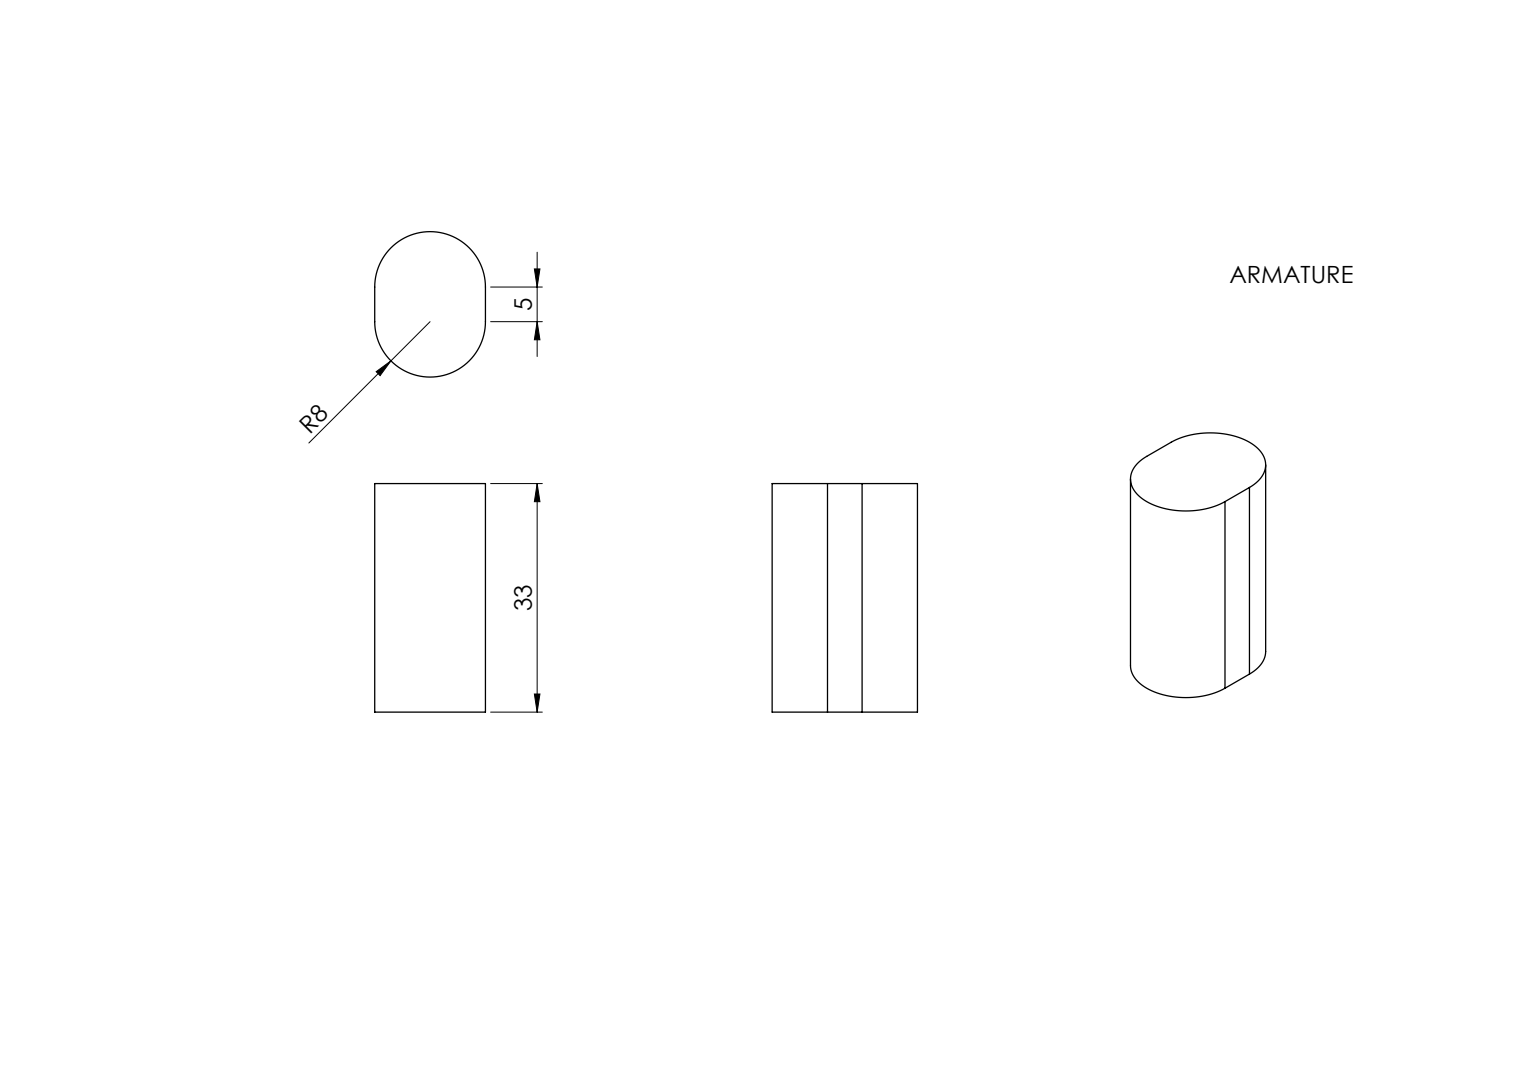
ISO-10303-21;
HEADER;
FILE_DESCRIPTION (('STEP AP214'),
    '1' );
FILE_NAME ('armature.step',
    '2026-10-25T16:39:07',
    ( '' ),
    ( '' ),
    'SwSTEP 2.0',
    'SolidWorks 2026',
    '' );
FILE_SCHEMA (( 'AUTOMOTIVE_DESIGN' ));
ENDSEC;

DATA;
#70=EDGE_LOOP ( 'NONE', ( #14455, #11089, #12235, #9427, #6688 ) ) ;
#196=VERTEX_POINT ( 'NONE', #13765 ) ;
#256=CARTESIAN_POINT ( 'NONE',  ( 7.960204194457794491E-16, 43.00000000000000000, 6.499999999999999112 ) ) ;
#309=AXIS2_PLACEMENT_3D ( 'NONE', #1703, #12902, #17104 ) ;
#401=CARTESIAN_POINT ( 'NONE',  ( 0.000000000000000000, 43.00000000000000000, -6.499999999999999112 ) ) ;
#459=( NAMED_UNIT ( * ) PLANE_ANGLE_UNIT ( ) SI_UNIT ( $, .RADIAN. ) );
#592=EDGE_CURVE ( 'NONE', #196, #11177, #4131, .T. ) ;
#631=EDGE_LOOP ( 'NONE', ( #5395, #16207, #13707, #2530 ) ) ;
#732=DIRECTION ( 'NONE',  ( 0.000000000000000000, 1.000000000000000000, 0.000000000000000000 ) ) ;
#736=DIRECTION ( 'NONE',  ( 0.000000000000000000, 0.000000000000000000, -1.000000000000000000 ) ) ;
#757=EDGE_LOOP ( 'NONE', ( #3139, #14699 ) ) ;
#760=FACE_OUTER_BOUND ( 'NONE', #70, .T. ) ;
#909=EDGE_CURVE ( 'NONE', #2259, #4661, #14792, .T. ) ;
#919=SURFACE_STYLE_USAGE ( .BOTH. , #14844 ) ;
#953=CIRCLE ( 'NONE', #984, 8.000000000000000000 ) ;
#956=( GEOMETRIC_REPRESENTATION_CONTEXT ( 3 ) GLOBAL_UNCERTAINTY_ASSIGNED_CONTEXT ( ( #17928 ) ) GLOBAL_UNIT_ASSIGNED_CONTEXT ( ( #7948, #17991, #15201 ) ) REPRESENTATION_CONTEXT ( 'NONE', 'WORKASPACE' ) );
#984=AXIS2_PLACEMENT_3D ( 'NONE', #4156, #12407, #11016 ) ;
#1007=DIRECTION ( 'NONE',  ( -0.000000000000000000, -1.000000000000000000, -0.000000000000000000 ) ) ;
#1011=ORIENTED_EDGE ( 'NONE', *, *, #17505, .F. ) ;
#1041=ORIENTED_EDGE ( 'NONE', *, *, #17682, .F. ) ;
#1082=LINE ( 'NONE', #2294, #16709 ) ;
#1153=DIRECTION ( 'NONE',  ( 0.000000000000000000, 1.000000000000000000, 0.000000000000000000 ) ) ;
#1197=DIRECTION ( 'NONE',  ( -3.469446951953612217E-16, 0.000000000000000000, -1.000000000000000000 ) ) ;
#1250=( GEOMETRIC_REPRESENTATION_CONTEXT ( 3 ) GLOBAL_UNCERTAINTY_ASSIGNED_CONTEXT ( ( #6593 ) ) GLOBAL_UNIT_ASSIGNED_CONTEXT ( ( #16139, #459, #11752 ) ) REPRESENTATION_CONTEXT ( 'NONE', 'WORKASPACE' ) );
#1394=CARTESIAN_POINT ( 'NONE',  ( 0.000000000000000000, 13.00000000000000178, 2.500000000000000000 ) ) ;
#1404=EDGE_CURVE ( 'NONE', #1787, #196, #16670, .T. ) ;
#1414=ORIENTED_EDGE ( 'NONE', *, *, #3097, .T. ) ;
#1509=ADVANCED_FACE ( 'NONE', ( #760, #4919 ), #10384, .F. ) ;
#1701=EDGE_CURVE ( 'NONE', #8991, #2259, #3048, .T. ) ;
#1703=CARTESIAN_POINT ( 'NONE',  ( 0.000000000000000000, 43.00000000000000000, 2.500000000000000000 ) ) ;
#1729=DIRECTION ( 'NONE',  ( 1.000000000000000000, 0.000000000000000000, -3.469446951953616654E-16 ) ) ;
#1787=VERTEX_POINT ( 'NONE', #17543 ) ;
#1846=CARTESIAN_POINT ( 'NONE',  ( -9.184850993605147944E-16, 13.00000000000000178, -2.500000000000000000 ) ) ;
#1918=DIRECTION ( 'NONE',  ( 0.000000000000000000, 0.000000000000000000, 1.000000000000000000 ) ) ;
#2259=VERTEX_POINT ( 'NONE', #3355 ) ;
#2294=CARTESIAN_POINT ( 'NONE',  ( 8.000000000000000000, 43.00000000000000000, 2.500000000000000000 ) ) ;
#2342=VERTEX_POINT ( 'NONE', #7514 ) ;
#2530=ORIENTED_EDGE ( 'NONE', *, *, #14666, .F. ) ;
#2571=VERTEX_POINT ( 'NONE', #8377 ) ;
#2643=AXIS2_PLACEMENT_3D ( 'NONE', #5642, #9539, #8055 ) ;
#2651=CARTESIAN_POINT ( 'NONE',  ( -9.184850993605147944E-16, 46.00000000000000000, -2.500000000000000000 ) ) ;
#2783=CARTESIAN_POINT ( 'NONE',  ( -9.184850993605147944E-16, 13.00000000000000178, -10.50000000000000000 ) ) ;
#2871=DIRECTION ( 'NONE',  ( 0.000000000000000000, 0.000000000000000000, 1.000000000000000000 ) ) ;
#2873=ADVANCED_FACE ( 'NONE', ( #5761 ), #8803, .T. ) ;
#3048=CIRCLE ( 'NONE', #11605, 8.000000000000000000 ) ;
#3054=CARTESIAN_POINT ( 'NONE',  ( -8.000000000000000000, 43.00000000000000000, 2.500000000000000000 ) ) ;
#3055=FILL_AREA_STYLE_COLOUR ( '', #3608 ) ;
#3097=EDGE_CURVE ( 'NONE', #11177, #2571, #18280, .T. ) ;
#3111=APPLICATION_CONTEXT ( 'automotive_design' ) ;
#3139=ORIENTED_EDGE ( 'NONE', *, *, #17076, .T. ) ;
#3211=PLANE ( 'NONE',  #6539 ) ;
#3302=DIRECTION ( 'NONE',  ( -3.469446951953616654E-16, 0.000000000000000000, -1.000000000000000000 ) ) ;
#3332=EDGE_CURVE ( 'NONE', #2342, #8991, #10075, .T. ) ;
#3355=CARTESIAN_POINT ( 'NONE',  ( 8.000000000000000000, 13.00000000000000178, 2.500000000000000000 ) ) ;
#3417=ADVANCED_BREP_SHAPE_REPRESENTATION ( '', ( #14274, #16940 ), #1250 ) ;
#3468=DIRECTION ( 'NONE',  ( -3.469446951953612217E-16, 0.000000000000000000, -1.000000000000000000 ) ) ;
#3608=COLOUR_RGB ( '',0.8941176470588234615, 0.8941176470588234615, 0.8941176470588234615 ) ;
#3751=DIRECTION ( 'NONE',  ( 3.469446951953612217E-16, 0.000000000000000000, 1.000000000000000000 ) ) ;
#3799=EDGE_LOOP ( 'NONE', ( #15244, #1011, #13623, #17796 ) ) ;
#3806=UNCERTAINTY_MEASURE_WITH_UNIT (LENGTH_MEASURE( 1.000000000000000082E-05 ), #14295, 'distance_accuracy_value', 'NONE');
#3912=VERTEX_POINT ( 'NONE', #4688 ) ;
#4006=SHAPE_REPRESENTATION ( 'armature', ( #16940 ), #1250 ) ;
#4131=CIRCLE ( 'NONE', #12999, 8.000000000000000000 ) ;
#4156=CARTESIAN_POINT ( 'NONE',  ( 0.000000000000000000, 46.00000000000000000, 2.500000000000000000 ) ) ;
#4157=AXIS2_PLACEMENT_3D ( 'NONE', #16906, #11305, #4182 ) ;
#4182=DIRECTION ( 'NONE',  ( 0.000000000000000000, 0.000000000000000000, -1.000000000000000000 ) ) ;
#4205=AXIS2_PLACEMENT_3D ( 'NONE', #10570, #17468, #10288 ) ;
#4206=LINE ( 'NONE', #11149, #15935 ) ;
#4431=CIRCLE ( 'NONE', #7691, 6.499999999999999112 ) ;
#4552=DIRECTION ( 'NONE',  ( 0.000000000000000000, 0.000000000000000000, 1.000000000000000000 ) ) ;
#4587=FACE_OUTER_BOUND ( 'NONE', #11356, .T. ) ;
#4661=VERTEX_POINT ( 'NONE', #10825 ) ;
#4688=CARTESIAN_POINT ( 'NONE',  ( 0.000000000000000000, 13.00000000000000178, -6.499999999999999112 ) ) ;
#4697=CIRCLE ( 'NONE', #2643, 6.499999999999999112 ) ;
#4731=EDGE_CURVE ( 'NONE', #12052, #1787, #8315, .T. ) ;
#4752=CIRCLE ( 'NONE', #11856, 6.499999999999999112 ) ;
#4869=ORIENTED_EDGE ( 'NONE', *, *, #10897, .T. ) ;
#4881=ORIENTED_EDGE ( 'NONE', *, *, #1404, .F. ) ;
#4919=FACE_BOUND ( 'NONE', #757, .T. ) ;
#5181=EDGE_CURVE ( 'NONE', #11177, #2342, #10621, .T. ) ;
#5247=EDGE_CURVE ( 'NONE', #12052, #2259, #1082, .T. ) ;
#5252=CARTESIAN_POINT ( 'NONE',  ( -8.000000000000001776, 46.00000000000000000, -2.500000000000000888 ) ) ;
#5263=SURFACE_STYLE_FILL_AREA ( #9519 ) ;
#5395=ORIENTED_EDGE ( 'NONE', *, *, #13177, .T. ) ;
#5591=EDGE_CURVE ( 'NONE', #2571, #8991, #9215, .T. ) ;
#5597=CARTESIAN_POINT ( 'NONE',  ( 8.000000000000000000, 46.00000000000000000, 2.500000000000000000 ) ) ;
#5642=CARTESIAN_POINT ( 'NONE',  ( 0.000000000000000000, 43.00000000000000000, 0.000000000000000000 ) ) ;
#5751=ADVANCED_FACE ( 'NONE', ( #11059 ), #18044, .T. ) ;
#5761=FACE_OUTER_BOUND ( 'NONE', #8478, .T. ) ;
#5974=EDGE_CURVE ( 'NONE', #14789, #7076, #15789, .T. ) ;
#6067=CARTESIAN_POINT ( 'NONE',  ( -8.000000000000000000, 43.00000000000000000, 2.500000000000000000 ) ) ;
#6090=DIRECTION ( 'NONE',  ( -0.000000000000000000, -1.000000000000000000, -0.000000000000000000 ) ) ;
#6283=ORIENTED_EDGE ( 'NONE', *, *, #1701, .T. ) ;
#6428=DIRECTION ( 'NONE',  ( 1.000000000000000000, 0.000000000000000000, 0.000000000000000000 ) ) ;
#6464=EDGE_LOOP ( 'NONE', ( #10886, #4881, #7225, #4869 ) ) ;
#6465=CARTESIAN_POINT ( 'NONE',  ( -9.184850993605147944E-16, 43.00000000000000000, -2.500000000000000000 ) ) ;
#6539=AXIS2_PLACEMENT_3D ( 'NONE', #6067, #1729, #3302 ) ;
#6593=UNCERTAINTY_MEASURE_WITH_UNIT (LENGTH_MEASURE( 1.000000000000000082E-05 ), #16139, 'distance_accuracy_value', 'NONE');
#6640=VERTEX_POINT ( 'NONE', #401 ) ;
#6688=ORIENTED_EDGE ( 'NONE', *, *, #909, .F. ) ;
#6693=ORIENTED_EDGE ( 'NONE', *, *, #5181, .T. ) ;
#6723=AXIS2_PLACEMENT_3D ( 'NONE', #12020, #6090, #10256 ) ;
#6892=DIRECTION ( 'NONE',  ( 0.000000000000000000, 1.000000000000000000, 0.000000000000000000 ) ) ;
#6917=ORIENTED_EDGE ( 'NONE', *, *, #8304, .T. ) ;
#7076=VERTEX_POINT ( 'NONE', #9078 ) ;
#7125=EDGE_LOOP ( 'NONE', ( #17051, #10261, #7653, #9888, #6693 ) ) ;
#7225=ORIENTED_EDGE ( 'NONE', *, *, #17505, .T. ) ;
#7226=EDGE_LOOP ( 'NONE', ( #10360, #14482, #7585, #16309 ) ) ;
#7293=CYLINDRICAL_SURFACE ( 'NONE', #14449, 6.499999999999999112 ) ;
#7320=EDGE_LOOP ( 'NONE', ( #13330, #1041 ) ) ;
#7386=ORIENTED_EDGE ( 'NONE', *, *, #5181, .F. ) ;
#7514=CARTESIAN_POINT ( 'NONE',  ( -8.000000000000000000, 46.00000000000000000, 2.499999999999999112 ) ) ;
#7585=ORIENTED_EDGE ( 'NONE', *, *, #14666, .T. ) ;
#7610=CIRCLE ( 'NONE', #17720, 8.000000000000000000 ) ;
#7625=EDGE_CURVE ( 'NONE', #7076, #3912, #4431, .T. ) ;
#7631=CLOSED_SHELL ( 'NONE', ( #17170, #17395, #1509, #2873, #13560, #10893, #17839, #13477, #16610, #5751 ) ) ;
#7635=DIRECTION ( 'NONE',  ( 0.000000000000000000, 1.000000000000000000, 0.000000000000000000 ) ) ;
#7653=ORIENTED_EDGE ( 'NONE', *, *, #1404, .T. ) ;
#7691=AXIS2_PLACEMENT_3D ( 'NONE', #16877, #12944, #14348 ) ;
#7819=CIRCLE ( 'NONE', #9592, 8.000000000000000000 ) ;
#7834=CARTESIAN_POINT ( 'NONE',  ( -8.000000000000000000, 46.00000000000000000, 2.499999999999999112 ) ) ;
#7946=ORIENTED_EDGE ( 'NONE', *, *, #592, .F. ) ;
#7948=( LENGTH_UNIT ( ) NAMED_UNIT ( * ) SI_UNIT ( .MILLI., .METRE. ) );
#7970=PRODUCT_DEFINITION_CONTEXT ( 'detailed design', #3111, 'design' ) ;
#8034=FACE_OUTER_BOUND ( 'NONE', #18065, .T. ) ;
#8050=AXIS2_PLACEMENT_3D ( 'NONE', #8528, #9920, #11311 ) ;
#8055=DIRECTION ( 'NONE',  ( 0.000000000000000000, 0.000000000000000000, 1.000000000000000000 ) ) ;
#8103=DIRECTION ( 'NONE',  ( 0.000000000000000000, 0.000000000000000000, 1.000000000000000000 ) ) ;
#8125=DIRECTION ( 'NONE',  ( -0.000000000000000000, -1.000000000000000000, -0.000000000000000000 ) ) ;
#8148=VECTOR ( 'NONE', #11143, 1000.000000000000000 ) ;
#8202=DIRECTION ( 'NONE',  ( -0.000000000000000000, -1.000000000000000000, -0.000000000000000000 ) ) ;
#8304=EDGE_CURVE ( 'NONE', #15374, #2571, #7819, .T. ) ;
#8315=LINE ( 'NONE', #15384, #10744 ) ;
#8377=CARTESIAN_POINT ( 'NONE',  ( -8.000000000000001776, 13.00000000000000178, -2.499999999999997335 ) ) ;
#8411=CARTESIAN_POINT ( 'NONE',  ( -8.000000000000000000, 13.00000000000000178, 2.500000000000000000 ) ) ;
#8478=EDGE_LOOP ( 'NONE', ( #6283, #14604, #16192, #16324 ) ) ;
#8524=ORIENTED_EDGE ( 'NONE', *, *, #3097, .F. ) ;
#8528=CARTESIAN_POINT ( 'NONE',  ( 0.000000000000000000, 43.00000000000000000, 2.500000000000000000 ) ) ;
#8683=DIRECTION ( 'NONE',  ( -0.000000000000000000, -1.000000000000000000, -0.000000000000000000 ) ) ;
#8717=CARTESIAN_POINT ( 'NONE',  ( 7.960204194457794491E-16, 43.00000000000000000, 6.499999999999999112 ) ) ;
#8774=EDGE_CURVE ( 'NONE', #2342, #12052, #953, .T. ) ;
#8803=CYLINDRICAL_SURFACE ( 'NONE', #8050, 8.000000000000000000 ) ;
#8928=MECHANICAL_DESIGN_GEOMETRIC_PRESENTATION_REPRESENTATION('',(#11896),#956);
#8991=VERTEX_POINT ( 'NONE', #8411 ) ;
#9004=( NAMED_UNIT ( * ) PLANE_ANGLE_UNIT ( ) SI_UNIT ( $, .RADIAN. ) );
#9024=CARTESIAN_POINT ( 'NONE',  ( 0.000000000000000000, 0.000000000000000000, 0.000000000000000000 ) ) ;
#9078=CARTESIAN_POINT ( 'NONE',  ( 7.960204194457794491E-16, 13.00000000000000178, 6.499999999999999112 ) ) ;
#9215=LINE ( 'NONE', #11707, #17622 ) ;
#9406=MECHANICAL_DESIGN_GEOMETRIC_PRESENTATION_REPRESENTATION('',(#15052),#11484);
#9427=ORIENTED_EDGE ( 'NONE', *, *, #10897, .F. ) ;
#9448=PRODUCT ( 'armature', 'armature', '', ( #17794 ) ) ;
#9492=FACE_OUTER_BOUND ( 'NONE', #3799, .T. ) ;
#9519=FILL_AREA_STYLE ('',( #3055 ) ) ;
#9539=DIRECTION ( 'NONE',  ( 0.000000000000000000, 1.000000000000000000, 0.000000000000000000 ) ) ;
#9585=AXIS2_PLACEMENT_3D ( 'NONE', #17778, #1153, #16741 ) ;
#9592=AXIS2_PLACEMENT_3D ( 'NONE', #15906, #7635, #1918 ) ;
#9691=CARTESIAN_POINT ( 'NONE',  ( 0.000000000000000000, 43.00000000000000000, 0.000000000000000000 ) ) ;
#9737=VECTOR ( 'NONE', #13895, 1000.000000000000000 ) ;
#9803=LINE ( 'NONE', #18097, #9737 ) ;
#9888=ORIENTED_EDGE ( 'NONE', *, *, #592, .T. ) ;
#9920=DIRECTION ( 'NONE',  ( -0.000000000000000000, -1.000000000000000000, -0.000000000000000000 ) ) ;
#10066=VECTOR ( 'NONE', #1007, 1000.000000000000000 ) ;
#10075=LINE ( 'NONE', #3054, #13388 ) ;
#10115=FACE_OUTER_BOUND ( 'NONE', #7320, .T. ) ;
#10256=DIRECTION ( 'NONE',  ( 0.000000000000000000, 0.000000000000000000, -1.000000000000000000 ) ) ;
#10260=DIRECTION ( 'NONE',  ( 0.000000000000000000, 0.000000000000000000, -1.000000000000000000 ) ) ;
#10261=ORIENTED_EDGE ( 'NONE', *, *, #4731, .T. ) ;
#10283=ORIENTED_EDGE ( 'NONE', *, *, #3332, .F. ) ;
#10288=DIRECTION ( 'NONE',  ( 0.000000000000000000, -0.000000000000000000, 1.000000000000000000 ) ) ;
#10309=CARTESIAN_POINT ( 'NONE',  ( 8.000000000000000000, 13.00000000000000178, 2.500000000000000000 ) ) ;
#10353=CYLINDRICAL_SURFACE ( 'NONE', #6723, 8.000000000000000000 ) ;
#10360=ORIENTED_EDGE ( 'NONE', *, *, #5974, .F. ) ;
#10384=PLANE ( 'NONE',  #4205 ) ;
#10570=CARTESIAN_POINT ( 'NONE',  ( 0.000000000000000000, 13.00000000000000178, 2.500000000000000000 ) ) ;
#10621=LINE ( 'NONE', #7834, #12524 ) ;
#10643=SHAPE_REPRESENTATION_RELATIONSHIP ( 'NONE' , 'NONE' ,  #4006, #3417 ) ;
#10711=ORIENTED_EDGE ( 'NONE', *, *, #5591, .T. ) ;
#10744=VECTOR ( 'NONE', #1197, 1000.000000000000000 ) ;
#10825=CARTESIAN_POINT ( 'NONE',  ( 7.999999999999998224, 13.00000000000000178, -2.500000000000003109 ) ) ;
#10841=DIRECTION ( 'NONE',  ( -0.000000000000000000, -1.000000000000000000, -0.000000000000000000 ) ) ;
#10886=ORIENTED_EDGE ( 'NONE', *, *, #12042, .F. ) ;
#10893=ADVANCED_FACE ( 'NONE', ( #13419 ), #10353, .T. ) ;
#10897=EDGE_CURVE ( 'NONE', #4661, #15374, #7610, .T. ) ;
#11016=DIRECTION ( 'NONE',  ( 0.000000000000000000, 0.000000000000000000, 1.000000000000000000 ) ) ;
#11059=FACE_OUTER_BOUND ( 'NONE', #7125, .T. ) ;
#11089=ORIENTED_EDGE ( 'NONE', *, *, #5591, .F. ) ;
#11143=DIRECTION ( 'NONE',  ( -0.000000000000000000, -1.000000000000000000, -0.000000000000000000 ) ) ;
#11149=CARTESIAN_POINT ( 'NONE',  ( -9.184850993605147944E-16, 43.00000000000000000, -10.50000000000000000 ) ) ;
#11177=VERTEX_POINT ( 'NONE', #5252 ) ;
#11244=DIRECTION ( 'NONE',  ( -0.000000000000000000, -1.000000000000000000, -0.000000000000000000 ) ) ;
#11305=DIRECTION ( 'NONE',  ( -0.000000000000000000, -1.000000000000000000, -0.000000000000000000 ) ) ;
#11311=DIRECTION ( 'NONE',  ( 0.000000000000000000, 0.000000000000000000, -1.000000000000000000 ) ) ;
#11356=EDGE_LOOP ( 'NONE', ( #10711, #10283, #7386, #1414 ) ) ;
#11392=CYLINDRICAL_SURFACE ( 'NONE', #4157, 6.499999999999999112 ) ;
#11456=AXIS2_PLACEMENT_3D ( 'NONE', #16469, #15170, #3751 ) ;
#11484=( GEOMETRIC_REPRESENTATION_CONTEXT ( 3 ) GLOBAL_UNCERTAINTY_ASSIGNED_CONTEXT ( ( #3806 ) ) GLOBAL_UNIT_ASSIGNED_CONTEXT ( ( #14295, #9004, #13261 ) ) REPRESENTATION_CONTEXT ( 'NONE', 'WORKASPACE' ) );
#11553=CIRCLE ( 'NONE', #16627, 6.499999999999999112 ) ;
#11595=AXIS2_PLACEMENT_3D ( 'NONE', #17281, #14678, #4552 ) ;
#11605=AXIS2_PLACEMENT_3D ( 'NONE', #1394, #15572, #2871 ) ;
#11695=PLANE ( 'NONE',  #309 ) ;
#11707=CARTESIAN_POINT ( 'NONE',  ( -8.000000000000000000, 13.00000000000000178, 2.500000000000000000 ) ) ;
#11752=( NAMED_UNIT ( * ) SI_UNIT ( $, .STERADIAN. ) SOLID_ANGLE_UNIT ( ) );
#11792=ORIENTED_EDGE ( 'NONE', *, *, #12042, .T. ) ;
#11856=AXIS2_PLACEMENT_3D ( 'NONE', #18215, #15421, #15142 ) ;
#11896=STYLED_ITEM ( 'NONE', ( #12029 ), #3417 ) ;
#11945=PRODUCT_DEFINITION ( 'UNKNOWN', '', #12792, #7970 ) ;
#12020=CARTESIAN_POINT ( 'NONE',  ( -9.184850993605147944E-16, 43.00000000000000000, -2.500000000000000000 ) ) ;
#12029=PRESENTATION_STYLE_ASSIGNMENT (( #919 ) ) ;
#12042=EDGE_CURVE ( 'NONE', #196, #15374, #4206, .T. ) ;
#12052=VERTEX_POINT ( 'NONE', #5597 ) ;
#12193=VECTOR ( 'NONE', #10841, 1000.000000000000000 ) ;
#12235=ORIENTED_EDGE ( 'NONE', *, *, #8304, .F. ) ;
#12407=DIRECTION ( 'NONE',  ( 0.000000000000000000, 1.000000000000000000, 0.000000000000000000 ) ) ;
#12524=VECTOR ( 'NONE', #17795, 1000.000000000000000 ) ;
#12792=PRODUCT_DEFINITION_FORMATION_WITH_SPECIFIED_SOURCE ( 'ANY', '', #9448, .NOT_KNOWN. ) ;
#12861=CARTESIAN_POINT ( 'NONE',  ( 0.000000000000000000, 43.00000000000000000, 0.000000000000000000 ) ) ;
#12902=DIRECTION ( 'NONE',  ( 0.000000000000000000, 1.000000000000000000, 0.000000000000000000 ) ) ;
#12944=DIRECTION ( 'NONE',  ( 0.000000000000000000, 1.000000000000000000, 0.000000000000000000 ) ) ;
#12999=AXIS2_PLACEMENT_3D ( 'NONE', #2651, #6892, #8103 ) ;
#13139=DIRECTION ( 'NONE',  ( 0.000000000000000000, 0.000000000000000000, 1.000000000000000000 ) ) ;
#13177=EDGE_CURVE ( 'NONE', #6640, #14789, #4697, .T. ) ;
#13261=( NAMED_UNIT ( * ) SI_UNIT ( $, .STERADIAN. ) SOLID_ANGLE_UNIT ( ) );
#13285=APPLICATION_CONTEXT ( 'automotive_design' ) ;
#13330=ORIENTED_EDGE ( 'NONE', *, *, #13177, .F. ) ;
#13388=VECTOR ( 'NONE', #8683, 1000.000000000000000 ) ;
#13419=FACE_OUTER_BOUND ( 'NONE', #6464, .T. ) ;
#13422=CYLINDRICAL_SURFACE ( 'NONE', #17216, 8.000000000000000000 ) ;
#13477=ADVANCED_FACE ( 'NONE', ( #14457 ), #7293, .F. ) ;
#13505=LINE ( 'NONE', #17892, #10066 ) ;
#13557=DIRECTION ( 'NONE',  ( 0.000000000000000000, 0.000000000000000000, 1.000000000000000000 ) ) ;
#13560=ADVANCED_FACE ( 'NONE', ( #9492 ), #16134, .F. ) ;
#13623=ORIENTED_EDGE ( 'NONE', *, *, #4731, .F. ) ;
#13707=ORIENTED_EDGE ( 'NONE', *, *, #17076, .F. ) ;
#13765=CARTESIAN_POINT ( 'NONE',  ( -9.184850993605147944E-16, 46.00000000000000000, -10.50000000000000000 ) ) ;
#13895=DIRECTION ( 'NONE',  ( -0.000000000000000000, -1.000000000000000000, -0.000000000000000000 ) ) ;
#14146=DIRECTION ( 'NONE',  ( 0.000000000000000000, 1.000000000000000000, 0.000000000000000000 ) ) ;
#14171=DIRECTION ( 'NONE',  ( -0.000000000000000000, -1.000000000000000000, -0.000000000000000000 ) ) ;
#14274=MANIFOLD_SOLID_BREP ( 'Boss-Extrude2', #7631 ) ;
#14295=( LENGTH_UNIT ( ) NAMED_UNIT ( * ) SI_UNIT ( .MILLI., .METRE. ) );
#14348=DIRECTION ( 'NONE',  ( 0.000000000000000000, 0.000000000000000000, 1.000000000000000000 ) ) ;
#14449=AXIS2_PLACEMENT_3D ( 'NONE', #12861, #14171, #10260 ) ;
#14455=ORIENTED_EDGE ( 'NONE', *, *, #1701, .F. ) ;
#14457=FACE_OUTER_BOUND ( 'NONE', #7226, .T. ) ;
#14482=ORIENTED_EDGE ( 'NONE', *, *, #17682, .T. ) ;
#14551=FACE_OUTER_BOUND ( 'NONE', #631, .T. ) ;
#14604=ORIENTED_EDGE ( 'NONE', *, *, #5247, .F. ) ;
#14666=EDGE_CURVE ( 'NONE', #6640, #3912, #9803, .T. ) ;
#14678=DIRECTION ( 'NONE',  ( 0.000000000000000000, 1.000000000000000000, 0.000000000000000000 ) ) ;
#14699=ORIENTED_EDGE ( 'NONE', *, *, #7625, .T. ) ;
#14789=VERTEX_POINT ( 'NONE', #256 ) ;
#14792=LINE ( 'NONE', #10309, #17504 ) ;
#14844=SURFACE_SIDE_STYLE ('',( #5263 ) ) ;
#15052=STYLED_ITEM('',(#18396),#14274);
#15142=DIRECTION ( 'NONE',  ( 0.000000000000000000, 0.000000000000000000, 1.000000000000000000 ) ) ;
#15170=DIRECTION ( 'NONE',  ( -1.000000000000000000, 0.000000000000000000, 3.469446951953612217E-16 ) ) ;
#15201=( NAMED_UNIT ( * ) SI_UNIT ( $, .STERADIAN. ) SOLID_ANGLE_UNIT ( ) );
#15244=ORIENTED_EDGE ( 'NONE', *, *, #909, .T. ) ;
#15374=VERTEX_POINT ( 'NONE', #2783 ) ;
#15384=CARTESIAN_POINT ( 'NONE',  ( 8.000000000000000000, 46.00000000000000000, 2.500000000000000000 ) ) ;
#15421=DIRECTION ( 'NONE',  ( 0.000000000000000000, 1.000000000000000000, 0.000000000000000000 ) ) ;
#15572=DIRECTION ( 'NONE',  ( 0.000000000000000000, 1.000000000000000000, 0.000000000000000000 ) ) ;
#15634=DIRECTION ( 'NONE',  ( 0.000000000000000000, 0.000000000000000000, 1.000000000000000000 ) ) ;
#15789=LINE ( 'NONE', #8717, #8148 ) ;
#15906=CARTESIAN_POINT ( 'NONE',  ( -9.184850993605147944E-16, 13.00000000000000178, -2.500000000000000000 ) ) ;
#15935=VECTOR ( 'NONE', #11244, 1000.000000000000000 ) ;
#16120=PRODUCT_DEFINITION_SHAPE ( 'NONE', 'NONE',  #11945 ) ;
#16134=PLANE ( 'NONE',  #11456 ) ;
#16139=( LENGTH_UNIT ( ) NAMED_UNIT ( * ) SI_UNIT ( .MILLI., .METRE. ) );
#16192=ORIENTED_EDGE ( 'NONE', *, *, #8774, .F. ) ;
#16207=ORIENTED_EDGE ( 'NONE', *, *, #5974, .T. ) ;
#16309=ORIENTED_EDGE ( 'NONE', *, *, #7625, .F. ) ;
#16324=ORIENTED_EDGE ( 'NONE', *, *, #3332, .T. ) ;
#16387=SHAPE_DEFINITION_REPRESENTATION ( #16120, #4006 ) ;
#16469=CARTESIAN_POINT ( 'NONE',  ( 8.000000000000000000, 43.00000000000000000, 2.500000000000000000 ) ) ;
#16610=ADVANCED_FACE ( 'NONE', ( #10115 ), #11695, .F. ) ;
#16627=AXIS2_PLACEMENT_3D ( 'NONE', #9691, #14146, #15634 ) ;
#16670=CIRCLE ( 'NONE', #11595, 8.000000000000000000 ) ;
#16709=VECTOR ( 'NONE', #8202, 1000.000000000000000 ) ;
#16741=DIRECTION ( 'NONE',  ( 0.000000000000000000, -0.000000000000000000, 1.000000000000000000 ) ) ;
#16799=CARTESIAN_POINT ( 'NONE',  ( -8.000000000000001776, 43.00000000000000000, -2.499999999999997335 ) ) ;
#16877=CARTESIAN_POINT ( 'NONE',  ( 0.000000000000000000, 13.00000000000000178, 0.000000000000000000 ) ) ;
#16906=CARTESIAN_POINT ( 'NONE',  ( 0.000000000000000000, 43.00000000000000000, 0.000000000000000000 ) ) ;
#16940=AXIS2_PLACEMENT_3D ( 'NONE', #9024, #13557, #6428 ) ;
#17051=ORIENTED_EDGE ( 'NONE', *, *, #8774, .T. ) ;
#17076=EDGE_CURVE ( 'NONE', #3912, #7076, #4752, .T. ) ;
#17104=DIRECTION ( 'NONE',  ( 0.000000000000000000, -0.000000000000000000, 1.000000000000000000 ) ) ;
#17170=ADVANCED_FACE ( 'NONE', ( #14551 ), #11392, .F. ) ;
#17216=AXIS2_PLACEMENT_3D ( 'NONE', #6465, #8125, #736 ) ;
#17281=CARTESIAN_POINT ( 'NONE',  ( -9.184850993605147944E-16, 46.00000000000000000, -2.500000000000000000 ) ) ;
#17395=ADVANCED_FACE ( 'NONE', ( #8034 ), #13422, .T. ) ;
#17468=DIRECTION ( 'NONE',  ( 0.000000000000000000, 1.000000000000000000, 0.000000000000000000 ) ) ;
#17498=DIRECTION ( 'NONE',  ( 3.469446951953616161E-16, -0.000000000000000000, 1.000000000000000000 ) ) ;
#17504=VECTOR ( 'NONE', #3468, 1000.000000000000000 ) ;
#17505=EDGE_CURVE ( 'NONE', #1787, #4661, #13505, .T. ) ;
#17543=CARTESIAN_POINT ( 'NONE',  ( 7.999999999999998224, 46.00000000000000000, -2.500000000000003109 ) ) ;
#17622=VECTOR ( 'NONE', #17498, 1000.000000000000000 ) ;
#17682=EDGE_CURVE ( 'NONE', #14789, #6640, #11553, .T. ) ;
#17720=AXIS2_PLACEMENT_3D ( 'NONE', #1846, #732, #13139 ) ;
#17778=CARTESIAN_POINT ( 'NONE',  ( 0.000000000000000000, 46.00000000000000000, 2.500000000000000000 ) ) ;
#17794=PRODUCT_CONTEXT ( 'NONE', #13285, 'mechanical' ) ;
#17795=DIRECTION ( 'NONE',  ( 3.469446951953614189E-16, -0.000000000000000000, 1.000000000000000000 ) ) ;
#17796=ORIENTED_EDGE ( 'NONE', *, *, #5247, .T. ) ;
#17839=ADVANCED_FACE ( 'NONE', ( #4587 ), #3211, .F. ) ;
#17892=CARTESIAN_POINT ( 'NONE',  ( 7.999999999999998224, 43.00000000000000000, -2.500000000000003109 ) ) ;
#17928=UNCERTAINTY_MEASURE_WITH_UNIT (LENGTH_MEASURE( 1.000000000000000082E-05 ), #7948, 'distance_accuracy_value', 'NONE');
#17991=( NAMED_UNIT ( * ) PLANE_ANGLE_UNIT ( ) SI_UNIT ( $, .RADIAN. ) );
#18044=PLANE ( 'NONE',  #9585 ) ;
#18065=EDGE_LOOP ( 'NONE', ( #7946, #11792, #6917, #8524 ) ) ;
#18097=CARTESIAN_POINT ( 'NONE',  ( 0.000000000000000000, 43.00000000000000000, -6.499999999999999112 ) ) ;
#18215=CARTESIAN_POINT ( 'NONE',  ( 0.000000000000000000, 13.00000000000000178, 0.000000000000000000 ) ) ;
#18280=LINE ( 'NONE', #16799, #12193 ) ;
#18390=COLOUR_RGB('Light Blue',0.38,0.62,0.78);
#18391=FILL_AREA_STYLE_COLOUR('',#18390);
#18392=FILL_AREA_STYLE('',(#18391));
#18393=SURFACE_STYLE_FILL_AREA(#18392);
#18394=SURFACE_SIDE_STYLE('',(#18393));
#18395=SURFACE_STYLE_USAGE(.BOTH.,#18394);
#18396=PRESENTATION_STYLE_ASSIGNMENT((#18395));
ENDSEC;
END-ISO-10303-21;
